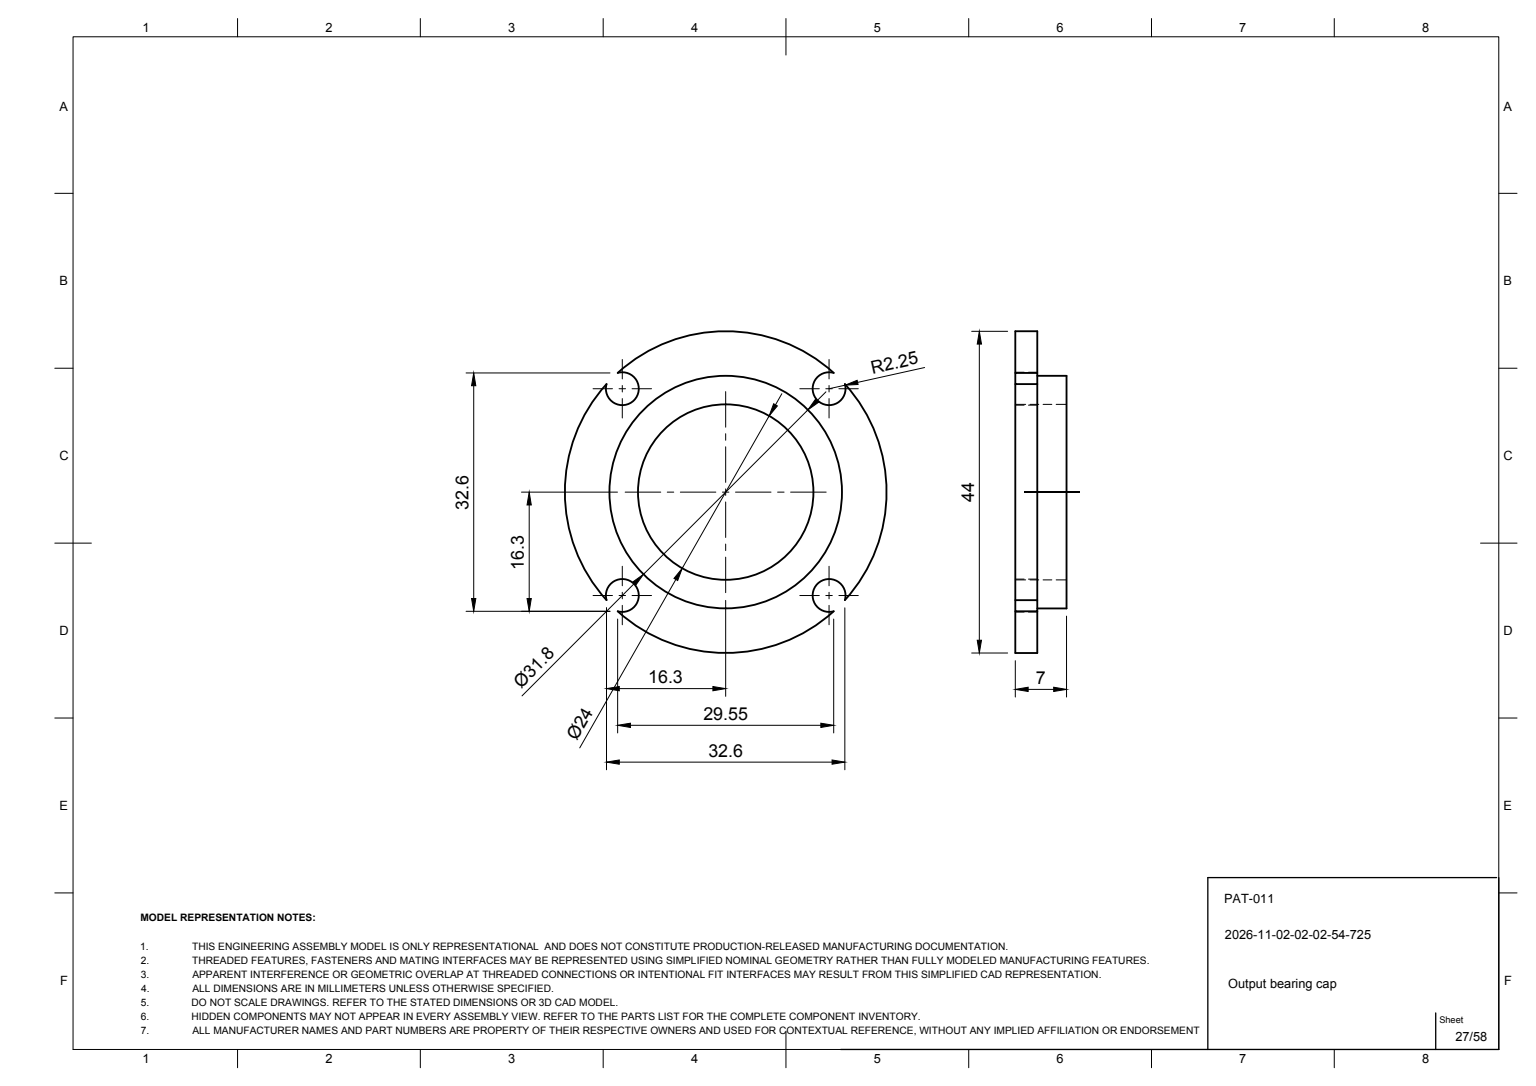
ISO-10303-21;
HEADER;
/* Generated by software containing ST-Developer
 * from STEP Tools, Inc. (www.steptools.com) 
 */

FILE_DESCRIPTION(
/* description */ ('Belt tension measurement rig'),
/* implementation_level */ '2;1');

FILE_NAME(
/* name */ 'Output bearing cap.step',
/* time_stamp */ '2026-10-28T03:24:44-07:00',
/* author */ (''),
/* organization */ (''),
/* preprocessor_version */ 'ST-DEVELOPER v20.2',
/* originating_system */ 'Autodesk Translation Framework v15.17.0.0',
/* authorisation */ '');

FILE_SCHEMA (('AUTOMOTIVE_DESIGN { 1 0 10303 214 3 1 1 }'));
ENDSEC;

DATA;
#10=MECHANICAL_DESIGN_GEOMETRIC_PRESENTATION_REPRESENTATION('',(#722),#23587);
#604=SHAPE_REPRESENTATION_RELATIONSHIP('SRR','None',#23851,#659);
#659=ADVANCED_BREP_SHAPE_REPRESENTATION('',(#792),#23549);
#722=STYLED_ITEM('',(#24211),#792);
#792=MANIFOLD_SOLID_BREP('Body1',#12227);
#956=FACE_BOUND('',#2463,.T.);
#957=FACE_BOUND('',#2470,.T.);
#958=FACE_BOUND('',#2473,.T.);
#1177=PLANE('',#13469);
#1178=PLANE('',#13486);
#1179=PLANE('',#13489);
#1627=FACE_OUTER_BOUND('',#2458,.T.);
#1628=FACE_OUTER_BOUND('',#2459,.T.);
#1629=FACE_OUTER_BOUND('',#2460,.T.);
#1630=FACE_OUTER_BOUND('',#2461,.T.);
#1631=FACE_OUTER_BOUND('',#2462,.T.);
#1632=FACE_OUTER_BOUND('',#2464,.T.);
#1633=FACE_OUTER_BOUND('',#2465,.T.);
#1634=FACE_OUTER_BOUND('',#2466,.T.);
#1635=FACE_OUTER_BOUND('',#2467,.T.);
#1636=FACE_OUTER_BOUND('',#2468,.T.);
#1637=FACE_OUTER_BOUND('',#2469,.T.);
#1638=FACE_OUTER_BOUND('',#2471,.T.);
#1639=FACE_OUTER_BOUND('',#2472,.T.);
#2458=EDGE_LOOP('',(#9142,#9143,#9144,#9145));
#2459=EDGE_LOOP('',(#9146,#9147,#9148,#9149));
#2460=EDGE_LOOP('',(#9150,#9151,#9152,#9153));
#2461=EDGE_LOOP('',(#9154,#9155,#9156,#9157));
#2462=EDGE_LOOP('',(#9158,#9159,#9160,#9161,#9162,#9163,#9164,#9165));
#2463=EDGE_LOOP('',(#9166));
#2464=EDGE_LOOP('',(#9167,#9168,#9169,#9170));
#2465=EDGE_LOOP('',(#9171,#9172,#9173,#9174));
#2466=EDGE_LOOP('',(#9175,#9176,#9177,#9178));
#2467=EDGE_LOOP('',(#9179,#9180,#9181,#9182));
#2468=EDGE_LOOP('',(#9183,#9184,#9185,#9186));
#2469=EDGE_LOOP('',(#9187));
#2470=EDGE_LOOP('',(#9188));
#2471=EDGE_LOOP('',(#9189,#9190,#9191,#9192));
#2472=EDGE_LOOP('',(#9193,#9194,#9195,#9196,#9197,#9198,#9199,#9200));
#2473=EDGE_LOOP('',(#9201));
#3274=LINE('',#20280,#4025);
#3275=LINE('',#20284,#4026);
#3276=LINE('',#20289,#4027);
#3277=LINE('',#20293,#4028);
#3278=LINE('',#20298,#4029);
#3279=LINE('',#20302,#4030);
#3280=LINE('',#20307,#4031);
#3281=LINE('',#20311,#4032);
#3282=LINE('',#20332,#4033);
#3283=LINE('',#20338,#4034);
#4025=VECTOR('',#15987,1.);
#4026=VECTOR('',#15990,1.);
#4027=VECTOR('',#15995,1.);
#4028=VECTOR('',#15998,1.);
#4029=VECTOR('',#16003,1.);
#4030=VECTOR('',#16006,1.);
#4031=VECTOR('',#16011,1.);
#4032=VECTOR('',#16014,1.);
#4033=VECTOR('',#16049,1.59);
#4034=VECTOR('',#16058,1.2);
#4744=CIRCLE('',#13458,0.225);
#4745=CIRCLE('',#13459,0.225);
#4746=CIRCLE('',#13461,0.225);
#4747=CIRCLE('',#13462,0.225);
#4748=CIRCLE('',#13464,0.225);
#4749=CIRCLE('',#13465,0.225);
#4750=CIRCLE('',#13467,0.225);
#4751=CIRCLE('',#13468,0.225);
#4752=CIRCLE('',#13470,2.2);
#4753=CIRCLE('',#13471,2.2);
#4754=CIRCLE('',#13472,2.2);
#4755=CIRCLE('',#13473,2.2);
#4756=CIRCLE('',#13474,1.2);
#4757=CIRCLE('',#13476,2.2);
#4758=CIRCLE('',#13478,2.2);
#4759=CIRCLE('',#13480,2.2);
#4760=CIRCLE('',#13482,2.2);
#4761=CIRCLE('',#13484,1.59);
#4762=CIRCLE('',#13485,1.59);
#4763=CIRCLE('',#13487,1.2);
#5646=VERTEX_POINT('',#20278);
#5647=VERTEX_POINT('',#20279);
#5648=VERTEX_POINT('',#20281);
#5649=VERTEX_POINT('',#20283);
#5650=VERTEX_POINT('',#20287);
#5651=VERTEX_POINT('',#20288);
#5652=VERTEX_POINT('',#20290);
#5653=VERTEX_POINT('',#20292);
#5654=VERTEX_POINT('',#20296);
#5655=VERTEX_POINT('',#20297);
#5656=VERTEX_POINT('',#20299);
#5657=VERTEX_POINT('',#20301);
#5658=VERTEX_POINT('',#20305);
#5659=VERTEX_POINT('',#20306);
#5660=VERTEX_POINT('',#20308);
#5661=VERTEX_POINT('',#20310);
#5662=VERTEX_POINT('',#20318);
#5663=VERTEX_POINT('',#20329);
#5664=VERTEX_POINT('',#20331);
#5665=VERTEX_POINT('',#20335);
#6930=EDGE_CURVE('',#5646,#5647,#3274,.T.);
#6931=EDGE_CURVE('',#5648,#5646,#4744,.T.);
#6932=EDGE_CURVE('',#5649,#5648,#3275,.T.);
#6933=EDGE_CURVE('',#5647,#5649,#4745,.T.);
#6934=EDGE_CURVE('',#5650,#5651,#3276,.T.);
#6935=EDGE_CURVE('',#5652,#5650,#4746,.T.);
#6936=EDGE_CURVE('',#5653,#5652,#3277,.T.);
#6937=EDGE_CURVE('',#5651,#5653,#4747,.T.);
#6938=EDGE_CURVE('',#5654,#5655,#3278,.T.);
#6939=EDGE_CURVE('',#5656,#5654,#4748,.T.);
#6940=EDGE_CURVE('',#5657,#5656,#3279,.T.);
#6941=EDGE_CURVE('',#5655,#5657,#4749,.T.);
#6942=EDGE_CURVE('',#5658,#5659,#3280,.T.);
#6943=EDGE_CURVE('',#5660,#5658,#4750,.T.);
#6944=EDGE_CURVE('',#5661,#5660,#3281,.T.);
#6945=EDGE_CURVE('',#5659,#5661,#4751,.T.);
#6946=EDGE_CURVE('',#5660,#5646,#4752,.T.);
#6947=EDGE_CURVE('',#5656,#5658,#4753,.T.);
#6948=EDGE_CURVE('',#5652,#5654,#4754,.T.);
#6949=EDGE_CURVE('',#5648,#5650,#4755,.T.);
#6950=EDGE_CURVE('',#5662,#5662,#4756,.T.);
#6951=EDGE_CURVE('',#5657,#5659,#4757,.T.);
#6952=EDGE_CURVE('',#5653,#5655,#4758,.T.);
#6953=EDGE_CURVE('',#5661,#5647,#4759,.T.);
#6954=EDGE_CURVE('',#5649,#5651,#4760,.T.);
#6955=EDGE_CURVE('',#5663,#5663,#4761,.T.);
#6956=EDGE_CURVE('',#5663,#5664,#3282,.T.);
#6957=EDGE_CURVE('',#5664,#5664,#4762,.T.);
#6958=EDGE_CURVE('',#5665,#5665,#4763,.T.);
#6959=EDGE_CURVE('',#5665,#5662,#3283,.T.);
#9142=ORIENTED_EDGE('',*,*,#6930,.F.);
#9143=ORIENTED_EDGE('',*,*,#6931,.F.);
#9144=ORIENTED_EDGE('',*,*,#6932,.F.);
#9145=ORIENTED_EDGE('',*,*,#6933,.F.);
#9146=ORIENTED_EDGE('',*,*,#6934,.F.);
#9147=ORIENTED_EDGE('',*,*,#6935,.F.);
#9148=ORIENTED_EDGE('',*,*,#6936,.F.);
#9149=ORIENTED_EDGE('',*,*,#6937,.F.);
#9150=ORIENTED_EDGE('',*,*,#6938,.F.);
#9151=ORIENTED_EDGE('',*,*,#6939,.F.);
#9152=ORIENTED_EDGE('',*,*,#6940,.F.);
#9153=ORIENTED_EDGE('',*,*,#6941,.F.);
#9154=ORIENTED_EDGE('',*,*,#6942,.F.);
#9155=ORIENTED_EDGE('',*,*,#6943,.F.);
#9156=ORIENTED_EDGE('',*,*,#6944,.F.);
#9157=ORIENTED_EDGE('',*,*,#6945,.F.);
#9158=ORIENTED_EDGE('',*,*,#6931,.T.);
#9159=ORIENTED_EDGE('',*,*,#6946,.F.);
#9160=ORIENTED_EDGE('',*,*,#6943,.T.);
#9161=ORIENTED_EDGE('',*,*,#6947,.F.);
#9162=ORIENTED_EDGE('',*,*,#6939,.T.);
#9163=ORIENTED_EDGE('',*,*,#6948,.F.);
#9164=ORIENTED_EDGE('',*,*,#6935,.T.);
#9165=ORIENTED_EDGE('',*,*,#6949,.F.);
#9166=ORIENTED_EDGE('',*,*,#6950,.F.);
#9167=ORIENTED_EDGE('',*,*,#6940,.T.);
#9168=ORIENTED_EDGE('',*,*,#6947,.T.);
#9169=ORIENTED_EDGE('',*,*,#6942,.T.);
#9170=ORIENTED_EDGE('',*,*,#6951,.F.);
#9171=ORIENTED_EDGE('',*,*,#6936,.T.);
#9172=ORIENTED_EDGE('',*,*,#6948,.T.);
#9173=ORIENTED_EDGE('',*,*,#6938,.T.);
#9174=ORIENTED_EDGE('',*,*,#6952,.F.);
#9175=ORIENTED_EDGE('',*,*,#6930,.T.);
#9176=ORIENTED_EDGE('',*,*,#6953,.F.);
#9177=ORIENTED_EDGE('',*,*,#6944,.T.);
#9178=ORIENTED_EDGE('',*,*,#6946,.T.);
#9179=ORIENTED_EDGE('',*,*,#6932,.T.);
#9180=ORIENTED_EDGE('',*,*,#6949,.T.);
#9181=ORIENTED_EDGE('',*,*,#6934,.T.);
#9182=ORIENTED_EDGE('',*,*,#6954,.F.);
#9183=ORIENTED_EDGE('',*,*,#6955,.F.);
#9184=ORIENTED_EDGE('',*,*,#6956,.T.);
#9185=ORIENTED_EDGE('',*,*,#6957,.F.);
#9186=ORIENTED_EDGE('',*,*,#6956,.F.);
#9187=ORIENTED_EDGE('',*,*,#6955,.T.);
#9188=ORIENTED_EDGE('',*,*,#6958,.T.);
#9189=ORIENTED_EDGE('',*,*,#6958,.F.);
#9190=ORIENTED_EDGE('',*,*,#6959,.T.);
#9191=ORIENTED_EDGE('',*,*,#6950,.T.);
#9192=ORIENTED_EDGE('',*,*,#6959,.F.);
#9193=ORIENTED_EDGE('',*,*,#6933,.T.);
#9194=ORIENTED_EDGE('',*,*,#6954,.T.);
#9195=ORIENTED_EDGE('',*,*,#6937,.T.);
#9196=ORIENTED_EDGE('',*,*,#6952,.T.);
#9197=ORIENTED_EDGE('',*,*,#6941,.T.);
#9198=ORIENTED_EDGE('',*,*,#6951,.T.);
#9199=ORIENTED_EDGE('',*,*,#6945,.T.);
#9200=ORIENTED_EDGE('',*,*,#6953,.T.);
#9201=ORIENTED_EDGE('',*,*,#6957,.T.);
#11271=CYLINDRICAL_SURFACE('',#13457,0.225);
#11272=CYLINDRICAL_SURFACE('',#13460,0.225);
#11273=CYLINDRICAL_SURFACE('',#13463,0.225);
#11274=CYLINDRICAL_SURFACE('',#13466,0.225);
#11275=CYLINDRICAL_SURFACE('',#13475,2.2);
#11276=CYLINDRICAL_SURFACE('',#13477,2.2);
#11277=CYLINDRICAL_SURFACE('',#13479,2.2);
#11278=CYLINDRICAL_SURFACE('',#13481,2.2);
#11279=CYLINDRICAL_SURFACE('',#13483,1.59);
#11280=CYLINDRICAL_SURFACE('',#13488,1.2);
#11768=ADVANCED_FACE('',(#1627),#11271,.F.);
#11769=ADVANCED_FACE('',(#1628),#11272,.F.);
#11770=ADVANCED_FACE('',(#1629),#11273,.F.);
#11771=ADVANCED_FACE('',(#1630),#11274,.F.);
#11772=ADVANCED_FACE('',(#1631,#956),#1177,.F.);
#11773=ADVANCED_FACE('',(#1632),#11275,.T.);
#11774=ADVANCED_FACE('',(#1633),#11276,.T.);
#11775=ADVANCED_FACE('',(#1634),#11277,.T.);
#11776=ADVANCED_FACE('',(#1635),#11278,.T.);
#11777=ADVANCED_FACE('',(#1636),#11279,.T.);
#11778=ADVANCED_FACE('',(#1637,#957),#1178,.T.);
#11779=ADVANCED_FACE('',(#1638),#11280,.F.);
#11780=ADVANCED_FACE('',(#1639,#958),#1179,.T.);
#12227=CLOSED_SHELL('',(#11768,#11769,#11770,#11771,#11772,#11773,#11774,
#11775,#11776,#11777,#11778,#11779,#11780));
#13456=AXIS2_PLACEMENT_3D('',#20276,#15983,#15984);
#13457=AXIS2_PLACEMENT_3D('',#20277,#15985,#15986);
#13458=AXIS2_PLACEMENT_3D('',#20282,#15988,#15989);
#13459=AXIS2_PLACEMENT_3D('',#20285,#15991,#15992);
#13460=AXIS2_PLACEMENT_3D('',#20286,#15993,#15994);
#13461=AXIS2_PLACEMENT_3D('',#20291,#15996,#15997);
#13462=AXIS2_PLACEMENT_3D('',#20294,#15999,#16000);
#13463=AXIS2_PLACEMENT_3D('',#20295,#16001,#16002);
#13464=AXIS2_PLACEMENT_3D('',#20300,#16004,#16005);
#13465=AXIS2_PLACEMENT_3D('',#20303,#16007,#16008);
#13466=AXIS2_PLACEMENT_3D('',#20304,#16009,#16010);
#13467=AXIS2_PLACEMENT_3D('',#20309,#16012,#16013);
#13468=AXIS2_PLACEMENT_3D('',#20312,#16015,#16016);
#13469=AXIS2_PLACEMENT_3D('',#20313,#16017,#16018);
#13470=AXIS2_PLACEMENT_3D('',#20314,#16019,#16020);
#13471=AXIS2_PLACEMENT_3D('',#20315,#16021,#16022);
#13472=AXIS2_PLACEMENT_3D('',#20316,#16023,#16024);
#13473=AXIS2_PLACEMENT_3D('',#20317,#16025,#16026);
#13474=AXIS2_PLACEMENT_3D('',#20319,#16027,#16028);
#13475=AXIS2_PLACEMENT_3D('',#20320,#16029,#16030);
#13476=AXIS2_PLACEMENT_3D('',#20321,#16031,#16032);
#13477=AXIS2_PLACEMENT_3D('',#20322,#16033,#16034);
#13478=AXIS2_PLACEMENT_3D('',#20323,#16035,#16036);
#13479=AXIS2_PLACEMENT_3D('',#20324,#16037,#16038);
#13480=AXIS2_PLACEMENT_3D('',#20325,#16039,#16040);
#13481=AXIS2_PLACEMENT_3D('',#20326,#16041,#16042);
#13482=AXIS2_PLACEMENT_3D('',#20327,#16043,#16044);
#13483=AXIS2_PLACEMENT_3D('',#20328,#16045,#16046);
#13484=AXIS2_PLACEMENT_3D('',#20330,#16047,#16048);
#13485=AXIS2_PLACEMENT_3D('',#20333,#16050,#16051);
#13486=AXIS2_PLACEMENT_3D('',#20334,#16052,#16053);
#13487=AXIS2_PLACEMENT_3D('',#20336,#16054,#16055);
#13488=AXIS2_PLACEMENT_3D('',#20337,#16056,#16057);
#13489=AXIS2_PLACEMENT_3D('',#20339,#16059,#16060);
#15983=DIRECTION('axis',(0.,0.,1.));
#15984=DIRECTION('refdir',(1.,0.,0.));
#15985=DIRECTION('center_axis',(0.,1.,0.));
#15986=DIRECTION('ref_axis',(0.707106781186549,0.,0.707106781186546));
#15987=DIRECTION('',(0.,1.,0.));
#15988=DIRECTION('center_axis',(0.,1.,0.));
#15989=DIRECTION('ref_axis',(1.,0.,0.));
#15990=DIRECTION('',(0.,-1.,0.));
#15991=DIRECTION('center_axis',(0.,-1.,0.));
#15992=DIRECTION('ref_axis',(1.,0.,0.));
#15993=DIRECTION('center_axis',(0.,1.,0.));
#15994=DIRECTION('ref_axis',(0.707106781186547,0.,-0.707106781186548));
#15995=DIRECTION('',(0.,1.,0.));
#15996=DIRECTION('center_axis',(0.,1.,0.));
#15997=DIRECTION('ref_axis',(1.,0.,0.));
#15998=DIRECTION('',(0.,-1.,0.));
#15999=DIRECTION('center_axis',(0.,-1.,0.));
#16000=DIRECTION('ref_axis',(1.,0.,0.));
#16001=DIRECTION('center_axis',(0.,1.,0.));
#16002=DIRECTION('ref_axis',(-0.707106781186548,0.,-0.707106781186547));
#16003=DIRECTION('',(0.,1.,0.));
#16004=DIRECTION('center_axis',(0.,1.,0.));
#16005=DIRECTION('ref_axis',(1.,0.,0.));
#16006=DIRECTION('',(0.,-1.,0.));
#16007=DIRECTION('center_axis',(0.,-1.,0.));
#16008=DIRECTION('ref_axis',(1.,0.,0.));
#16009=DIRECTION('center_axis',(0.,1.,0.));
#16010=DIRECTION('ref_axis',(-0.707106781186552,0.,0.707106781186543));
#16011=DIRECTION('',(0.,1.,0.));
#16012=DIRECTION('center_axis',(0.,1.,0.));
#16013=DIRECTION('ref_axis',(1.,0.,0.));
#16014=DIRECTION('',(0.,-1.,0.));
#16015=DIRECTION('center_axis',(0.,-1.,0.));
#16016=DIRECTION('ref_axis',(1.,0.,0.));
#16017=DIRECTION('center_axis',(0.,1.,0.));
#16018=DIRECTION('ref_axis',(1.,0.,0.));
#16019=DIRECTION('center_axis',(0.,1.,0.));
#16020=DIRECTION('ref_axis',(1.,0.,0.));
#16021=DIRECTION('center_axis',(0.,1.,0.));
#16022=DIRECTION('ref_axis',(1.,0.,0.));
#16023=DIRECTION('center_axis',(0.,1.,0.));
#16024=DIRECTION('ref_axis',(1.,0.,0.));
#16025=DIRECTION('center_axis',(0.,1.,0.));
#16026=DIRECTION('ref_axis',(1.,0.,0.));
#16027=DIRECTION('center_axis',(0.,-1.,0.));
#16028=DIRECTION('ref_axis',(1.,0.,0.));
#16029=DIRECTION('center_axis',(0.,1.,0.));
#16030=DIRECTION('ref_axis',(1.,0.,0.));
#16031=DIRECTION('center_axis',(0.,1.,0.));
#16032=DIRECTION('ref_axis',(1.,0.,0.));
#16033=DIRECTION('center_axis',(0.,1.,0.));
#16034=DIRECTION('ref_axis',(1.,0.,0.));
#16035=DIRECTION('center_axis',(0.,1.,0.));
#16036=DIRECTION('ref_axis',(1.,0.,0.));
#16037=DIRECTION('center_axis',(0.,1.,0.));
#16038=DIRECTION('ref_axis',(1.,0.,0.));
#16039=DIRECTION('center_axis',(0.,1.,0.));
#16040=DIRECTION('ref_axis',(1.,0.,0.));
#16041=DIRECTION('center_axis',(0.,1.,0.));
#16042=DIRECTION('ref_axis',(-1.,0.,-1.22464679914735E-16));
#16043=DIRECTION('center_axis',(0.,1.,0.));
#16044=DIRECTION('ref_axis',(1.,0.,0.));
#16045=DIRECTION('center_axis',(0.,1.,0.));
#16046=DIRECTION('ref_axis',(1.,0.,0.));
#16047=DIRECTION('center_axis',(0.,1.,0.));
#16048=DIRECTION('ref_axis',(1.,0.,0.));
#16049=DIRECTION('',(0.,-1.,0.));
#16050=DIRECTION('center_axis',(0.,-1.,0.));
#16051=DIRECTION('ref_axis',(1.,0.,0.));
#16052=DIRECTION('center_axis',(0.,1.,0.));
#16053=DIRECTION('ref_axis',(1.,0.,0.));
#16054=DIRECTION('center_axis',(0.,-1.,0.));
#16055=DIRECTION('ref_axis',(1.,0.,0.));
#16056=DIRECTION('center_axis',(0.,1.,0.));
#16057=DIRECTION('ref_axis',(1.,0.,0.));
#16058=DIRECTION('',(0.,-1.,0.));
#16059=DIRECTION('center_axis',(0.,1.,0.));
#16060=DIRECTION('ref_axis',(1.,0.,0.));
#20276=CARTESIAN_POINT('',(0.,0.,0.));
#20277=CARTESIAN_POINT('Origin',(8.5857864376269,-2.2,5.58578643762691));
#20278=CARTESIAN_POINT('',(8.52266468006184,-2.1,5.3698219874924));
#20279=CARTESIAN_POINT('',(8.52266468006184,-1.8,5.3698219874924));
#20280=CARTESIAN_POINT('',(8.52266468006184,-2.2,5.3698219874924));
#20281=CARTESIAN_POINT('',(8.3698219874924,-2.1,5.52266468006184));
#20282=CARTESIAN_POINT('Origin',(8.5857864376269,-2.1,5.58578643762691));
#20283=CARTESIAN_POINT('',(8.3698219874924,-1.8,5.52266468006184));
#20284=CARTESIAN_POINT('',(8.3698219874924,-2.2,5.52266468006184));
#20285=CARTESIAN_POINT('Origin',(8.5857864376269,-1.8,5.58578643762691));
#20286=CARTESIAN_POINT('Origin',(8.5857864376269,-2.2,8.4142135623731));
#20287=CARTESIAN_POINT('',(8.3698219874924,-2.1,8.47733531993816));
#20288=CARTESIAN_POINT('',(8.3698219874924,-1.8,8.47733531993816));
#20289=CARTESIAN_POINT('',(8.3698219874924,-2.2,8.47733531993816));
#20290=CARTESIAN_POINT('',(8.52266468006184,-2.1,8.6301780125076));
#20291=CARTESIAN_POINT('Origin',(8.5857864376269,-2.1,8.4142135623731));
#20292=CARTESIAN_POINT('',(8.52266468006184,-1.8,8.6301780125076));
#20293=CARTESIAN_POINT('',(8.52266468006184,-2.2,8.6301780125076));
#20294=CARTESIAN_POINT('Origin',(8.5857864376269,-1.8,8.4142135623731));
#20295=CARTESIAN_POINT('Origin',(11.4142135623731,-2.2,8.4142135623731));
#20296=CARTESIAN_POINT('',(11.4773353199382,-2.1,8.6301780125076));
#20297=CARTESIAN_POINT('',(11.4773353199382,-1.8,8.6301780125076));
#20298=CARTESIAN_POINT('',(11.4773353199382,-2.2,8.6301780125076));
#20299=CARTESIAN_POINT('',(11.6301780125076,-2.1,8.47733531993816));
#20300=CARTESIAN_POINT('Origin',(11.4142135623731,-2.1,8.4142135623731));
#20301=CARTESIAN_POINT('',(11.6301780125076,-1.8,8.47733531993816));
#20302=CARTESIAN_POINT('',(11.6301780125076,-2.2,8.47733531993816));
#20303=CARTESIAN_POINT('Origin',(11.4142135623731,-1.8,8.4142135623731));
#20304=CARTESIAN_POINT('Origin',(11.4142135623731,-2.2,5.58578643762691));
#20305=CARTESIAN_POINT('',(11.6301780125076,-2.1,5.52266468006184));
#20306=CARTESIAN_POINT('',(11.6301780125076,-1.8,5.52266468006184));
#20307=CARTESIAN_POINT('',(11.6301780125076,-2.2,5.52266468006184));
#20308=CARTESIAN_POINT('',(11.4773353199382,-2.1,5.3698219874924));
#20309=CARTESIAN_POINT('Origin',(11.4142135623731,-2.1,5.58578643762691));
#20310=CARTESIAN_POINT('',(11.4773353199382,-1.8,5.3698219874924));
#20311=CARTESIAN_POINT('',(11.4773353199382,-2.2,5.3698219874924));
#20312=CARTESIAN_POINT('Origin',(11.4142135623731,-1.8,5.58578643762691));
#20313=CARTESIAN_POINT('Origin',(10.,-2.1,7.));
#20314=CARTESIAN_POINT('Origin',(10.,-2.1,7.));
#20315=CARTESIAN_POINT('Origin',(10.,-2.1,7.));
#20316=CARTESIAN_POINT('Origin',(10.,-2.1,7.));
#20317=CARTESIAN_POINT('Origin',(10.,-2.1,7.));
#20318=CARTESIAN_POINT('',(8.8,-2.1,7.));
#20319=CARTESIAN_POINT('Origin',(10.,-2.1,7.));
#20320=CARTESIAN_POINT('Origin',(10.,-2.1,7.));
#20321=CARTESIAN_POINT('Origin',(10.,-1.8,7.));
#20322=CARTESIAN_POINT('Origin',(10.,-2.1,7.));
#20323=CARTESIAN_POINT('Origin',(10.,-1.8,7.));
#20324=CARTESIAN_POINT('Origin',(10.,-2.1,7.));
#20325=CARTESIAN_POINT('Origin',(10.,-1.8,7.));
#20326=CARTESIAN_POINT('Origin',(10.,-2.1,7.));
#20327=CARTESIAN_POINT('Origin',(10.,-1.8,7.));
#20328=CARTESIAN_POINT('Origin',(10.,-1.8,7.));
#20329=CARTESIAN_POINT('',(8.41,-1.4,7.));
#20330=CARTESIAN_POINT('Origin',(10.,-1.4,7.));
#20331=CARTESIAN_POINT('',(8.41,-1.8,7.));
#20332=CARTESIAN_POINT('',(8.41,-1.8,7.));
#20333=CARTESIAN_POINT('Origin',(10.,-1.8,7.));
#20334=CARTESIAN_POINT('Origin',(10.,-1.4,7.));
#20335=CARTESIAN_POINT('',(8.8,-1.4,7.));
#20336=CARTESIAN_POINT('Origin',(10.,-1.4,7.));
#20337=CARTESIAN_POINT('Origin',(10.,-2.1,7.));
#20338=CARTESIAN_POINT('',(8.8,-2.1,7.));
#20339=CARTESIAN_POINT('Origin',(10.,-1.8,7.));
#23484=UNCERTAINTY_MEASURE_WITH_UNIT(LENGTH_MEASURE(0.001),#23588,
'DISTANCE_ACCURACY_VALUE',
'Maximum model space distance between geometric entities at asserted c
onnectivities');
#23522=UNCERTAINTY_MEASURE_WITH_UNIT(LENGTH_MEASURE(0.001),#23588,
'DISTANCE_ACCURACY_VALUE',
'Maximum model space distance between geometric entities at asserted c
onnectivities');
#23549=(
GEOMETRIC_REPRESENTATION_CONTEXT(3)
GLOBAL_UNCERTAINTY_ASSIGNED_CONTEXT((#23484))
GLOBAL_UNIT_ASSIGNED_CONTEXT((#23588,#23590,#23591))
REPRESENTATION_CONTEXT('','3D')
);
#23587=(
GEOMETRIC_REPRESENTATION_CONTEXT(3)
GLOBAL_UNCERTAINTY_ASSIGNED_CONTEXT((#23522))
GLOBAL_UNIT_ASSIGNED_CONTEXT((#23588,#23590,#23591))
REPRESENTATION_CONTEXT('','3D')
);
#23588=(
LENGTH_UNIT()
NAMED_UNIT(*)
SI_UNIT(.CENTI.,.METRE.)
);
#23590=(
NAMED_UNIT(*)
PLANE_ANGLE_UNIT()
SI_UNIT($,.RADIAN.)
);
#23591=(
NAMED_UNIT(*)
SI_UNIT($,.STERADIAN.)
SOLID_ANGLE_UNIT()
);
#23618=SHAPE_DEFINITION_REPRESENTATION(#23687,#23851);
#23687=PRODUCT_DEFINITION_SHAPE('',$,#23916);
#23851=SHAPE_REPRESENTATION('',(#13456),#23549);
#23889=PRODUCT_DEFINITION_CONTEXT('part definition',#24083,'design');
#23916=PRODUCT_DEFINITION('Output bearing cap','Output bearing cap',#23980,
#23889);
#23980=PRODUCT_DEFINITION_FORMATION('',$,#24111);
#24083=APPLICATION_CONTEXT(
'Core Data for Automotive Mechanical Design Process');
#24084=PRODUCT_CONTEXT('part definition',#24083,'mechanical');
#24111=PRODUCT('Output bearing cap','Output bearing cap',
'Output bearing cap',(#24084));
#24205=COLOUR_RGB('Grey',0.48,0.52,0.57);
#24206=FILL_AREA_STYLE_COLOUR('',#24205);
#24207=FILL_AREA_STYLE('',(#24206));
#24208=SURFACE_STYLE_FILL_AREA(#24207);
#24209=SURFACE_SIDE_STYLE('',(#24208));
#24210=SURFACE_STYLE_USAGE(.BOTH.,#24209);
#24211=PRESENTATION_STYLE_ASSIGNMENT((#24210));
ENDSEC;
END-ISO-10303-21;
